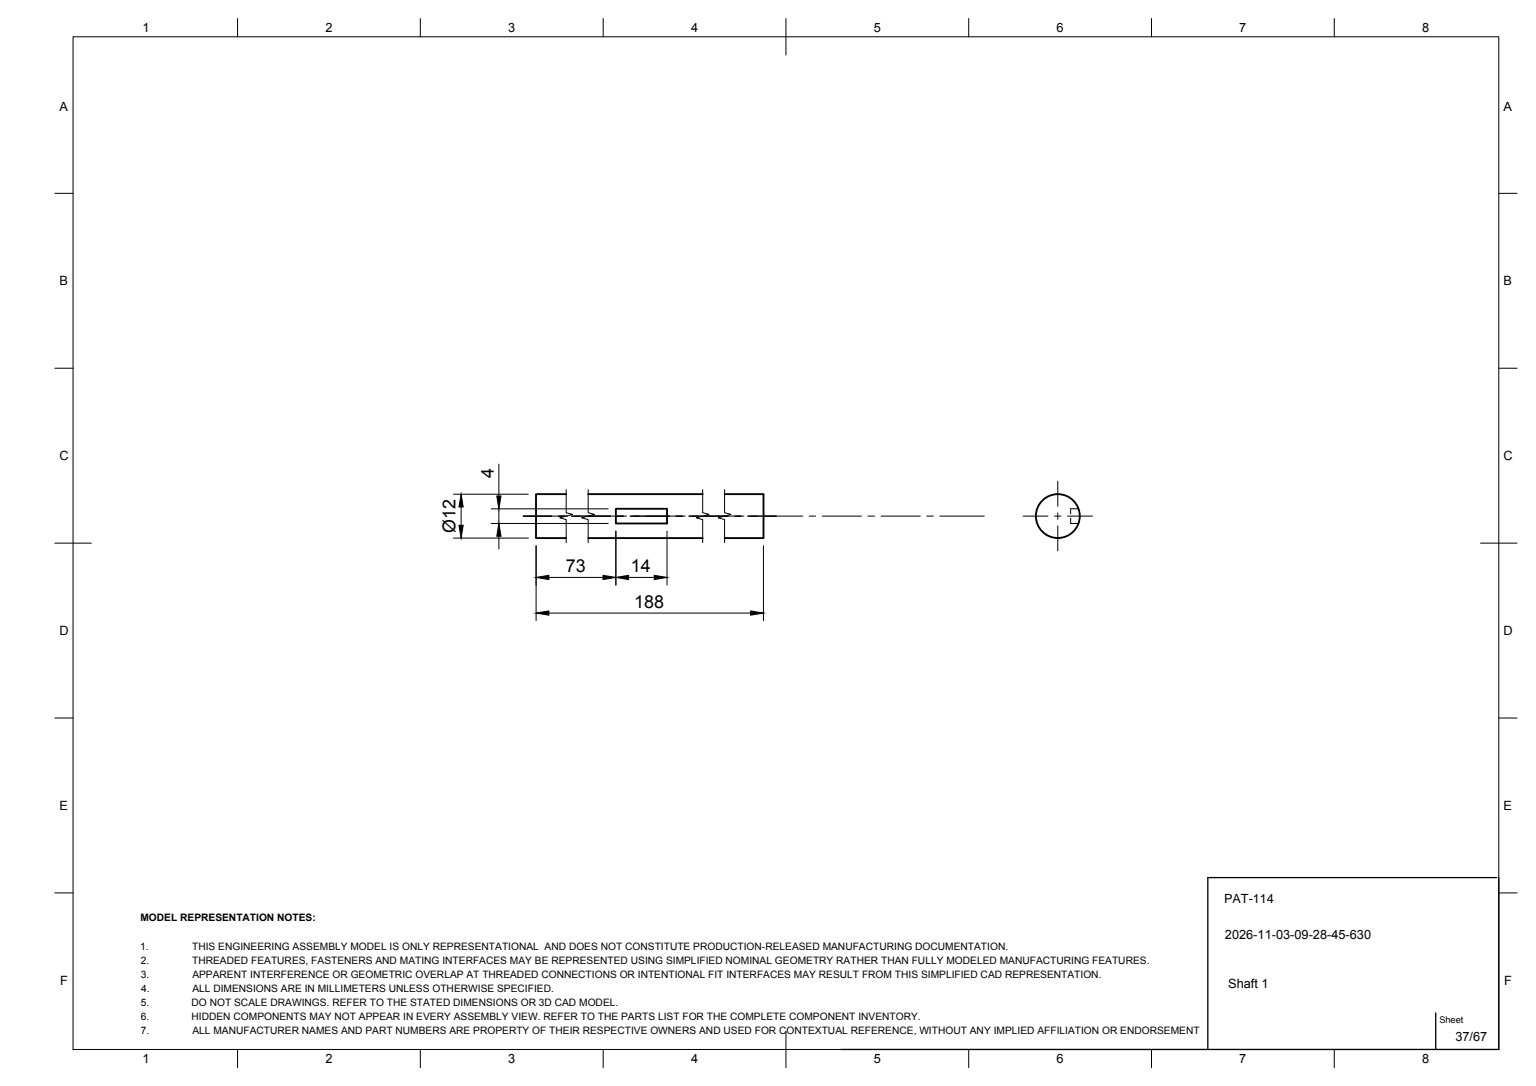
ISO-10303-21;
HEADER;
/* Generated by software containing ST-Developer
 * from STEP Tools, Inc. (www.steptools.com) 
 */

FILE_DESCRIPTION(
/* description */ ('Two-stage gear reducer in split housing'),
/* implementation_level */ '2;1');

FILE_NAME(
/* name */ 'Shaft 1.step',
/* time_stamp */ '2026-10-28T03:22:31-07:00',
/* author */ (''),
/* organization */ (''),
/* preprocessor_version */ 'ST-DEVELOPER v20.2',
/* originating_system */ 'Autodesk Translation Framework v15.17.0.0',
/* authorisation */ '');

FILE_SCHEMA (('AUTOMOTIVE_DESIGN { 1 0 10303 214 3 1 1 }'));
ENDSEC;

DATA;
#10=MECHANICAL_DESIGN_GEOMETRIC_PRESENTATION_REPRESENTATION('',(#1277),#73366);
#1150=SHAPE_REPRESENTATION_RELATIONSHIP('SRR','None',#73640,#1206);
#1206=ADVANCED_BREP_SHAPE_REPRESENTATION('',(#1346),#73336);
#1277=STYLED_ITEM('',(#73988),#1346);
#1346=MANIFOLD_SOLID_BREP('Body1',#16167);
#1538=FACE_BOUND('',#3499,.T.);
#1799=PLANE('',#17766);
#1800=PLANE('',#17767);
#1801=PLANE('',#17769);
#1802=PLANE('',#17770);
#1803=PLANE('',#17771);
#1804=PLANE('',#17776);
#1805=PLANE('',#17777);
#2416=FACE_OUTER_BOUND('',#3493,.T.);
#2417=FACE_OUTER_BOUND('',#3494,.T.);
#2418=FACE_OUTER_BOUND('',#3495,.T.);
#2419=FACE_OUTER_BOUND('',#3496,.T.);
#2420=FACE_OUTER_BOUND('',#3497,.T.);
#2421=FACE_OUTER_BOUND('',#3498,.T.);
#2422=FACE_OUTER_BOUND('',#3500,.T.);
#2423=FACE_OUTER_BOUND('',#3501,.T.);
#3493=EDGE_LOOP('',(#12289,#12290,#12291,#12292));
#3494=EDGE_LOOP('',(#12293,#12294,#12295,#12296));
#3495=EDGE_LOOP('',(#12297,#12298,#12299,#12300));
#3496=EDGE_LOOP('',(#12301,#12302,#12303,#12304));
#3497=EDGE_LOOP('',(#12305,#12306,#12307,#12308));
#3498=EDGE_LOOP('',(#12309,#12310,#12311,#12312));
#3499=EDGE_LOOP('',(#12313,#12314,#12315,#12316));
#3500=EDGE_LOOP('',(#12317));
#3501=EDGE_LOOP('',(#12318));
#4479=LINE('',#25427,#5503);
#4480=LINE('',#25429,#5504);
#4481=LINE('',#25431,#5505);
#4482=LINE('',#25432,#5506);
#4483=LINE('',#25437,#5507);
#4484=LINE('',#25438,#5508);
#4485=LINE('',#25441,#5509);
#4486=LINE('',#25443,#5510);
#4487=LINE('',#25444,#5511);
#4488=LINE('',#25446,#5512);
#4489=LINE('',#25453,#5513);
#5503=VECTOR('',#20791,1.);
#5504=VECTOR('',#20792,1.);
#5505=VECTOR('',#20793,1.);
#5506=VECTOR('',#20794,1.);
#5507=VECTOR('',#20799,1.);
#5508=VECTOR('',#20800,1.);
#5509=VECTOR('',#20803,1.);
#5510=VECTOR('',#20804,1.);
#5511=VECTOR('',#20805,1.);
#5512=VECTOR('',#20808,1.);
#5513=VECTOR('',#20817,0.6);
#6540=CIRCLE('',#17768,0.6);
#6541=CIRCLE('',#17772,0.6);
#6542=CIRCLE('',#17774,0.6);
#6543=CIRCLE('',#17775,0.6);
#7433=VERTEX_POINT('',#25425);
#7434=VERTEX_POINT('',#25426);
#7435=VERTEX_POINT('',#25428);
#7436=VERTEX_POINT('',#25430);
#7437=VERTEX_POINT('',#25434);
#7438=VERTEX_POINT('',#25436);
#7439=VERTEX_POINT('',#25440);
#7440=VERTEX_POINT('',#25442);
#7441=VERTEX_POINT('',#25450);
#7442=VERTEX_POINT('',#25452);
#9198=EDGE_CURVE('',#7433,#7434,#4479,.T.);
#9199=EDGE_CURVE('',#7433,#7435,#4480,.T.);
#9200=EDGE_CURVE('',#7436,#7435,#4481,.T.);
#9201=EDGE_CURVE('',#7436,#7434,#4482,.T.);
#9202=EDGE_CURVE('',#7434,#7437,#6540,.T.);
#9203=EDGE_CURVE('',#7438,#7436,#4483,.T.);
#9204=EDGE_CURVE('',#7437,#7438,#4484,.T.);
#9205=EDGE_CURVE('',#7437,#7439,#4485,.T.);
#9206=EDGE_CURVE('',#7438,#7440,#4486,.T.);
#9207=EDGE_CURVE('',#7440,#7439,#4487,.T.);
#9208=EDGE_CURVE('',#7435,#7440,#4488,.T.);
#9209=EDGE_CURVE('',#7439,#7433,#6541,.T.);
#9210=EDGE_CURVE('',#7441,#7441,#6542,.T.);
#9211=EDGE_CURVE('',#7441,#7442,#4489,.T.);
#9212=EDGE_CURVE('',#7442,#7442,#6543,.T.);
#12289=ORIENTED_EDGE('',*,*,#9198,.F.);
#12290=ORIENTED_EDGE('',*,*,#9199,.T.);
#12291=ORIENTED_EDGE('',*,*,#9200,.F.);
#12292=ORIENTED_EDGE('',*,*,#9201,.T.);
#12293=ORIENTED_EDGE('',*,*,#9202,.F.);
#12294=ORIENTED_EDGE('',*,*,#9201,.F.);
#12295=ORIENTED_EDGE('',*,*,#9203,.F.);
#12296=ORIENTED_EDGE('',*,*,#9204,.F.);
#12297=ORIENTED_EDGE('',*,*,#9205,.F.);
#12298=ORIENTED_EDGE('',*,*,#9204,.T.);
#12299=ORIENTED_EDGE('',*,*,#9206,.T.);
#12300=ORIENTED_EDGE('',*,*,#9207,.T.);
#12301=ORIENTED_EDGE('',*,*,#9203,.T.);
#12302=ORIENTED_EDGE('',*,*,#9200,.T.);
#12303=ORIENTED_EDGE('',*,*,#9208,.T.);
#12304=ORIENTED_EDGE('',*,*,#9206,.F.);
#12305=ORIENTED_EDGE('',*,*,#9209,.F.);
#12306=ORIENTED_EDGE('',*,*,#9207,.F.);
#12307=ORIENTED_EDGE('',*,*,#9208,.F.);
#12308=ORIENTED_EDGE('',*,*,#9199,.F.);
#12309=ORIENTED_EDGE('',*,*,#9210,.F.);
#12310=ORIENTED_EDGE('',*,*,#9211,.T.);
#12311=ORIENTED_EDGE('',*,*,#9212,.T.);
#12312=ORIENTED_EDGE('',*,*,#9211,.F.);
#12313=ORIENTED_EDGE('',*,*,#9205,.T.);
#12314=ORIENTED_EDGE('',*,*,#9209,.T.);
#12315=ORIENTED_EDGE('',*,*,#9198,.T.);
#12316=ORIENTED_EDGE('',*,*,#9202,.T.);
#12317=ORIENTED_EDGE('',*,*,#9210,.T.);
#12318=ORIENTED_EDGE('',*,*,#9212,.F.);
#15075=CYLINDRICAL_SURFACE('',#17773,0.6);
#15623=ADVANCED_FACE('',(#2416),#1799,.F.);
#15624=ADVANCED_FACE('',(#2417),#1800,.T.);
#15625=ADVANCED_FACE('',(#2418),#1801,.F.);
#15626=ADVANCED_FACE('',(#2419),#1802,.F.);
#15627=ADVANCED_FACE('',(#2420),#1803,.F.);
#15628=ADVANCED_FACE('',(#2421,#1538),#15075,.T.);
#15629=ADVANCED_FACE('',(#2422),#1804,.T.);
#15630=ADVANCED_FACE('',(#2423),#1805,.F.);
#16167=CLOSED_SHELL('',(#15623,#15624,#15625,#15626,#15627,#15628,#15629,
#15630));
#17765=AXIS2_PLACEMENT_3D('',#25423,#20787,#20788);
#17766=AXIS2_PLACEMENT_3D('',#25424,#20789,#20790);
#17767=AXIS2_PLACEMENT_3D('',#25433,#20795,#20796);
#17768=AXIS2_PLACEMENT_3D('',#25435,#20797,#20798);
#17769=AXIS2_PLACEMENT_3D('',#25439,#20801,#20802);
#17770=AXIS2_PLACEMENT_3D('',#25445,#20806,#20807);
#17771=AXIS2_PLACEMENT_3D('',#25447,#20809,#20810);
#17772=AXIS2_PLACEMENT_3D('',#25448,#20811,#20812);
#17773=AXIS2_PLACEMENT_3D('',#25449,#20813,#20814);
#17774=AXIS2_PLACEMENT_3D('',#25451,#20815,#20816);
#17775=AXIS2_PLACEMENT_3D('',#25454,#20818,#20819);
#17776=AXIS2_PLACEMENT_3D('',#25455,#20820,#20821);
#17777=AXIS2_PLACEMENT_3D('',#25456,#20822,#20823);
#20787=DIRECTION('axis',(0.,0.,1.));
#20788=DIRECTION('refdir',(1.,0.,0.));
#20789=DIRECTION('center_axis',(-1.,0.,0.));
#20790=DIRECTION('ref_axis',(0.,0.,1.));
#20791=DIRECTION('',(0.,-1.,0.));
#20792=DIRECTION('',(0.,0.,1.));
#20793=DIRECTION('',(0.,1.,0.));
#20794=DIRECTION('',(0.,0.,-1.));
#20795=DIRECTION('center_axis',(0.,1.,0.));
#20796=DIRECTION('ref_axis',(1.,0.,0.));
#20797=DIRECTION('center_axis',(0.,-1.,0.));
#20798=DIRECTION('ref_axis',(1.,0.,0.));
#20799=DIRECTION('',(-1.,0.,0.));
#20800=DIRECTION('',(0.,0.,1.));
#20801=DIRECTION('center_axis',(1.,0.,0.));
#20802=DIRECTION('ref_axis',(0.,0.,-1.));
#20803=DIRECTION('',(0.,1.,0.));
#20804=DIRECTION('',(0.,1.,0.));
#20805=DIRECTION('',(0.,0.,-1.));
#20806=DIRECTION('center_axis',(0.,0.,1.));
#20807=DIRECTION('ref_axis',(1.,0.,0.));
#20808=DIRECTION('',(1.,0.,0.));
#20809=DIRECTION('center_axis',(0.,1.,0.));
#20810=DIRECTION('ref_axis',(0.,0.,1.));
#20811=DIRECTION('center_axis',(0.,1.,0.));
#20812=DIRECTION('ref_axis',(1.,0.,0.));
#20813=DIRECTION('center_axis',(0.,1.,0.));
#20814=DIRECTION('ref_axis',(1.,0.,0.));
#20815=DIRECTION('center_axis',(0.,1.,0.));
#20816=DIRECTION('ref_axis',(1.,0.,0.));
#20817=DIRECTION('',(0.,-1.,0.));
#20818=DIRECTION('center_axis',(0.,1.,0.));
#20819=DIRECTION('ref_axis',(1.,0.,0.));
#20820=DIRECTION('center_axis',(0.,1.,0.));
#20821=DIRECTION('ref_axis',(1.,0.,0.));
#20822=DIRECTION('center_axis',(0.,1.,0.));
#20823=DIRECTION('ref_axis',(1.,0.,0.));
#25423=CARTESIAN_POINT('',(0.,0.,0.));
#25424=CARTESIAN_POINT('Origin',(-0.2,-2.1,8.8));
#25425=CARTESIAN_POINT('',(-0.2,-0.699999999999999,9.43431457505076));
#25426=CARTESIAN_POINT('',(-0.2,-2.1,9.43431457505076));
#25427=CARTESIAN_POINT('',(-0.2,-9.4,9.43431457505076));
#25428=CARTESIAN_POINT('',(-0.2,-0.7,9.65));
#25429=CARTESIAN_POINT('',(-0.2,-0.7,9.65));
#25430=CARTESIAN_POINT('',(-0.2,-2.1,9.65));
#25431=CARTESIAN_POINT('',(-0.2,-2.1,9.65));
#25432=CARTESIAN_POINT('',(-0.2,-2.1,9.65));
#25433=CARTESIAN_POINT('Origin',(0.,-2.1,9.225));
#25434=CARTESIAN_POINT('',(0.2,-2.1,9.43431457505076));
#25435=CARTESIAN_POINT('Origin',(0.,-2.1,10.));
#25436=CARTESIAN_POINT('',(0.2,-2.1,9.65));
#25437=CARTESIAN_POINT('',(0.2,-2.1,9.65));
#25438=CARTESIAN_POINT('',(0.2,-2.1,8.8));
#25439=CARTESIAN_POINT('Origin',(0.2,-2.1,9.65));
#25440=CARTESIAN_POINT('',(0.2,-0.699999999999999,9.43431457505076));
#25441=CARTESIAN_POINT('',(0.2,-9.4,9.43431457505076));
#25442=CARTESIAN_POINT('',(0.2,-0.7,9.65));
#25443=CARTESIAN_POINT('',(0.2,-2.1,9.65));
#25444=CARTESIAN_POINT('',(0.2,-0.7,8.8));
#25445=CARTESIAN_POINT('Origin',(-0.2,-2.1,9.65));
#25446=CARTESIAN_POINT('',(0.2,-0.7,9.65));
#25447=CARTESIAN_POINT('Origin',(0.,-0.7,9.225));
#25448=CARTESIAN_POINT('Origin',(0.,-0.699999999999999,10.));
#25449=CARTESIAN_POINT('Origin',(0.,-9.4,10.));
#25450=CARTESIAN_POINT('',(-0.6,9.4,10.));
#25451=CARTESIAN_POINT('Origin',(0.,9.4,10.));
#25452=CARTESIAN_POINT('',(-0.6,-9.4,10.));
#25453=CARTESIAN_POINT('',(-0.6,-9.4,10.));
#25454=CARTESIAN_POINT('Origin',(0.,-9.4,10.));
#25455=CARTESIAN_POINT('Origin',(0.,9.4,10.));
#25456=CARTESIAN_POINT('Origin',(0.,-9.4,10.));
#73272=UNCERTAINTY_MEASURE_WITH_UNIT(LENGTH_MEASURE(0.001),#73367,
'DISTANCE_ACCURACY_VALUE',
'Maximum model space distance between geometric entities at asserted c
onnectivities');
#73302=UNCERTAINTY_MEASURE_WITH_UNIT(LENGTH_MEASURE(0.001),#73367,
'DISTANCE_ACCURACY_VALUE',
'Maximum model space distance between geometric entities at asserted c
onnectivities');
#73336=(
GEOMETRIC_REPRESENTATION_CONTEXT(3)
GLOBAL_UNCERTAINTY_ASSIGNED_CONTEXT((#73272))
GLOBAL_UNIT_ASSIGNED_CONTEXT((#73367,#73369,#73370))
REPRESENTATION_CONTEXT('','3D')
);
#73366=(
GEOMETRIC_REPRESENTATION_CONTEXT(3)
GLOBAL_UNCERTAINTY_ASSIGNED_CONTEXT((#73302))
GLOBAL_UNIT_ASSIGNED_CONTEXT((#73367,#73369,#73370))
REPRESENTATION_CONTEXT('','3D')
);
#73367=(
LENGTH_UNIT()
NAMED_UNIT(*)
SI_UNIT(.CENTI.,.METRE.)
);
#73369=(
NAMED_UNIT(*)
PLANE_ANGLE_UNIT()
SI_UNIT($,.RADIAN.)
);
#73370=(
NAMED_UNIT(*)
SI_UNIT($,.STERADIAN.)
SOLID_ANGLE_UNIT()
);
#73404=SHAPE_DEFINITION_REPRESENTATION(#73537,#73640);
#73537=PRODUCT_DEFINITION_SHAPE('',$,#73704);
#73640=SHAPE_REPRESENTATION('',(#17765),#73336);
#73670=PRODUCT_DEFINITION_CONTEXT('part definition',#73861,'design');
#73704=PRODUCT_DEFINITION('Shaft 1','Shaft 1',#73767,#73670);
#73767=PRODUCT_DEFINITION_FORMATION('',$,#73896);
#73861=APPLICATION_CONTEXT(
'Core Data for Automotive Mechanical Design Process');
#73862=PRODUCT_CONTEXT('part definition',#73861,'mechanical');
#73896=PRODUCT('Shaft 1','Shaft 1','Shaft 1',(#73862));
#73982=COLOUR_RGB('Grey',0.48,0.52,0.57);
#73983=FILL_AREA_STYLE_COLOUR('',#73982);
#73984=FILL_AREA_STYLE('',(#73983));
#73985=SURFACE_STYLE_FILL_AREA(#73984);
#73986=SURFACE_SIDE_STYLE('',(#73985));
#73987=SURFACE_STYLE_USAGE(.BOTH.,#73986);
#73988=PRESENTATION_STYLE_ASSIGNMENT((#73987));
ENDSEC;
END-ISO-10303-21;
